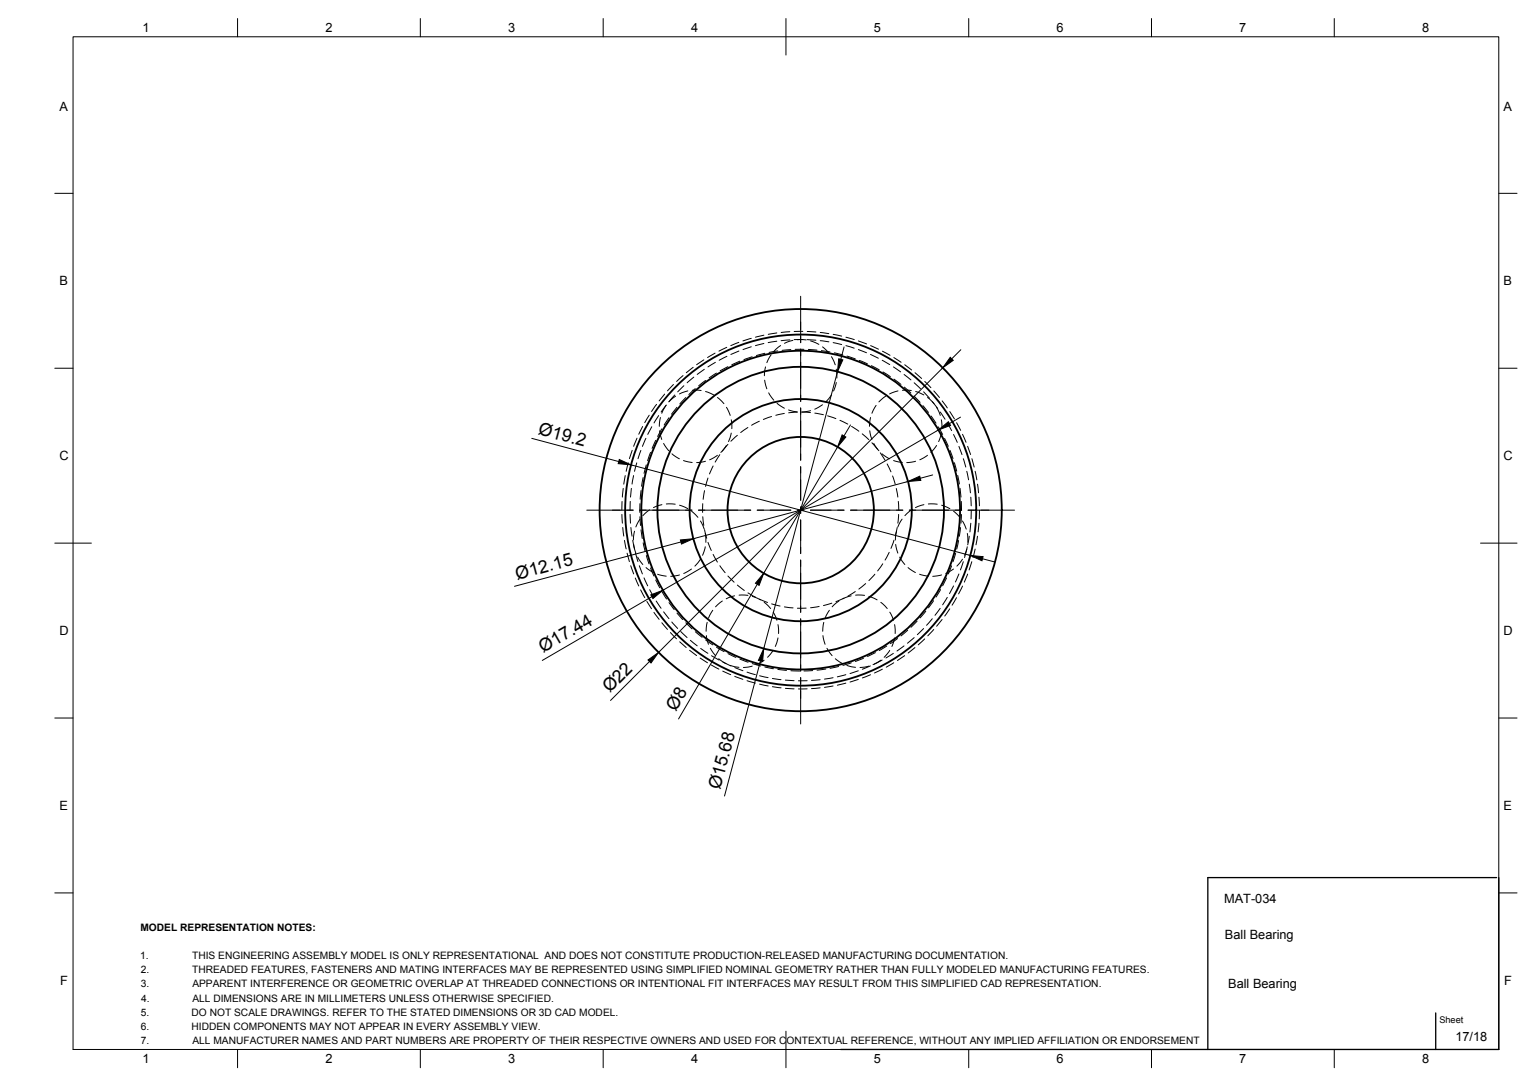
ISO-10303-21;
HEADER;
/* Generated by software containing ST-Developer
 * from STEP Tools, Inc. (www.steptools.com) 
 */

FILE_DESCRIPTION(
/* description */ ('STEP AP214'),
/* implementation_level */ '2;1');

FILE_NAME(
/* name */ 'Ball Bearing.step',
/* time_stamp */ '2026-11-14T09:24:36-08:00',
/* author */ (''),
/* organization */ (''),
/* preprocessor_version */ 'ST-DEVELOPER v20.2',
/* originating_system */ 'Autodesk Translation Framework v15.17.0.0',
/* authorisation */ '');

FILE_SCHEMA (('AUTOMOTIVE_DESIGN { 1 0 10303 214 3 1 1 }'));
ENDSEC;

DATA;
#10=MECHANICAL_DESIGN_GEOMETRIC_PRESENTATION_REPRESENTATION('',(#218,#219,#220,#221,#222,#223,#224,#225,#226),#18867);
#123=SPHERICAL_SURFACE('',#12164,1.9845);
#124=SPHERICAL_SURFACE('',#12166,1.9845);
#125=SPHERICAL_SURFACE('',#12168,1.9845);
#126=SPHERICAL_SURFACE('',#12170,1.9845);
#127=SPHERICAL_SURFACE('',#12172,1.9845);
#128=SPHERICAL_SURFACE('',#12174,1.9845);
#129=SPHERICAL_SURFACE('',#12176,1.9845);
#132=CONICAL_SURFACE('',#12193,8.8,1.39626340159546);
#133=CONICAL_SURFACE('',#12203,9.6,1.39626340159547);
#134=CONICAL_SURFACE('',#12217,9.6,1.46902152746005);
#135=CONICAL_SURFACE('',#12222,8.71875,1.51977681092793);
#136=CONICAL_SURFACE('',#12225,7.8375,1.51977681092793);
#137=CONICAL_SURFACE('',#12227,7.8375,1.51977681092793);
#138=CONICAL_SURFACE('',#12231,8.71875,1.46902152746005);
#139=CONICAL_SURFACE('',#12235,6.075,1.51977681092793);
#140=CONICAL_SURFACE('',#12238,8.71875,1.51977681092792);
#141=CONICAL_SURFACE('',#12242,9.6,1.51977681092792);
#157=TOROIDAL_SURFACE('',#12178,10.7,0.3);
#158=TOROIDAL_SURFACE('',#12184,10.7,0.3);
#159=TOROIDAL_SURFACE('',#12190,9.6,0.18);
#160=TOROIDAL_SURFACE('',#12197,7.35,1.9845);
#161=TOROIDAL_SURFACE('',#12206,9.6,0.18);
#162=TOROIDAL_SURFACE('',#12213,7.35,1.9845);
#163=TOROIDAL_SURFACE('',#12250,5.975,0.1);
#164=TOROIDAL_SURFACE('',#12253,4.3,0.3);
#165=TOROIDAL_SURFACE('',#12259,4.3,0.3);
#166=TOROIDAL_SURFACE('',#12262,5.975,0.1);
#186=SHAPE_REPRESENTATION_RELATIONSHIP('SRR','None',#18950,#202);
#202=ADVANCED_BREP_SHAPE_REPRESENTATION('',(#242,#243,#244,#245,#246,#247,
#248,#249,#250),#18866);
#218=STYLED_ITEM('',(#19027),#242);
#219=STYLED_ITEM('',(#19027),#243);
#220=STYLED_ITEM('',(#19027),#244);
#221=STYLED_ITEM('',(#19027),#245);
#222=STYLED_ITEM('',(#19027),#246);
#223=STYLED_ITEM('',(#19027),#247);
#224=STYLED_ITEM('',(#19027),#248);
#225=STYLED_ITEM('',(#19027),#249);
#226=STYLED_ITEM('',(#19027),#250);
#242=MANIFOLD_SOLID_BREP('Body1',#10973);
#243=MANIFOLD_SOLID_BREP('Body2',#10974);
#244=MANIFOLD_SOLID_BREP('Body3',#10975);
#245=MANIFOLD_SOLID_BREP('Body4',#10976);
#246=MANIFOLD_SOLID_BREP('Body5',#10977);
#247=MANIFOLD_SOLID_BREP('Body6',#10978);
#248=MANIFOLD_SOLID_BREP('Body7',#10979);
#249=MANIFOLD_SOLID_BREP('Body8',#10980);
#250=MANIFOLD_SOLID_BREP('Body9',#10981);
#373=FACE_BOUND('',#2012,.T.);
#374=FACE_BOUND('',#2014,.T.);
#375=FACE_BOUND('',#2036,.T.);
#376=FACE_BOUND('',#2038,.T.);
#377=FACE_BOUND('',#2040,.T.);
#378=FACE_BOUND('',#2042,.T.);
#379=FACE_BOUND('',#2044,.T.);
#380=FACE_BOUND('',#2046,.T.);
#717=PLANE('',#12211);
#718=PLANE('',#12212);
#719=PLANE('',#12269);
#720=PLANE('',#12270);
#721=PLANE('',#12271);
#722=PLANE('',#12272);
#723=PLANE('',#12273);
#724=PLANE('',#12274);
#1274=FACE_OUTER_BOUND('',#1992,.T.);
#1275=FACE_OUTER_BOUND('',#1993,.T.);
#1276=FACE_OUTER_BOUND('',#1994,.T.);
#1277=FACE_OUTER_BOUND('',#1995,.T.);
#1278=FACE_OUTER_BOUND('',#1996,.T.);
#1279=FACE_OUTER_BOUND('',#1997,.T.);
#1280=FACE_OUTER_BOUND('',#1998,.T.);
#1281=FACE_OUTER_BOUND('',#1999,.T.);
#1282=FACE_OUTER_BOUND('',#2000,.T.);
#1283=FACE_OUTER_BOUND('',#2001,.T.);
#1284=FACE_OUTER_BOUND('',#2002,.T.);
#1285=FACE_OUTER_BOUND('',#2003,.T.);
#1286=FACE_OUTER_BOUND('',#2004,.T.);
#1287=FACE_OUTER_BOUND('',#2005,.T.);
#1288=FACE_OUTER_BOUND('',#2006,.T.);
#1289=FACE_OUTER_BOUND('',#2007,.T.);
#1290=FACE_OUTER_BOUND('',#2008,.T.);
#1291=FACE_OUTER_BOUND('',#2009,.T.);
#1292=FACE_OUTER_BOUND('',#2010,.T.);
#1293=FACE_OUTER_BOUND('',#2011,.T.);
#1294=FACE_OUTER_BOUND('',#2013,.T.);
#1295=FACE_OUTER_BOUND('',#2015,.T.);
#1296=FACE_OUTER_BOUND('',#2016,.T.);
#1297=FACE_OUTER_BOUND('',#2017,.T.);
#1298=FACE_OUTER_BOUND('',#2018,.T.);
#1299=FACE_OUTER_BOUND('',#2019,.T.);
#1300=FACE_OUTER_BOUND('',#2020,.T.);
#1301=FACE_OUTER_BOUND('',#2021,.T.);
#1302=FACE_OUTER_BOUND('',#2022,.T.);
#1303=FACE_OUTER_BOUND('',#2023,.T.);
#1304=FACE_OUTER_BOUND('',#2024,.T.);
#1305=FACE_OUTER_BOUND('',#2025,.T.);
#1306=FACE_OUTER_BOUND('',#2026,.T.);
#1307=FACE_OUTER_BOUND('',#2027,.T.);
#1308=FACE_OUTER_BOUND('',#2028,.T.);
#1309=FACE_OUTER_BOUND('',#2029,.T.);
#1310=FACE_OUTER_BOUND('',#2030,.T.);
#1311=FACE_OUTER_BOUND('',#2031,.T.);
#1312=FACE_OUTER_BOUND('',#2032,.T.);
#1313=FACE_OUTER_BOUND('',#2033,.T.);
#1314=FACE_OUTER_BOUND('',#2034,.T.);
#1315=FACE_OUTER_BOUND('',#2035,.T.);
#1316=FACE_OUTER_BOUND('',#2037,.T.);
#1317=FACE_OUTER_BOUND('',#2039,.T.);
#1318=FACE_OUTER_BOUND('',#2041,.T.);
#1319=FACE_OUTER_BOUND('',#2043,.T.);
#1320=FACE_OUTER_BOUND('',#2045,.T.);
#1992=EDGE_LOOP('',(#9978,#9979));
#1993=EDGE_LOOP('',(#9980,#9981));
#1994=EDGE_LOOP('',(#9982,#9983));
#1995=EDGE_LOOP('',(#9984,#9985));
#1996=EDGE_LOOP('',(#9986,#9987));
#1997=EDGE_LOOP('',(#9988,#9989));
#1998=EDGE_LOOP('',(#9990,#9991));
#1999=EDGE_LOOP('',(#9992,#9993,#9994,#9995));
#2000=EDGE_LOOP('',(#9996,#9997,#9998,#9999));
#2001=EDGE_LOOP('',(#10000,#10001,#10002,#10003));
#2002=EDGE_LOOP('',(#10004,#10005,#10006,#10007));
#2003=EDGE_LOOP('',(#10008,#10009,#10010,#10011));
#2004=EDGE_LOOP('',(#10012,#10013,#10014,#10015));
#2005=EDGE_LOOP('',(#10016,#10017,#10018,#10019));
#2006=EDGE_LOOP('',(#10020,#10021,#10022,#10023));
#2007=EDGE_LOOP('',(#10024,#10025,#10026,#10027,#10028));
#2008=EDGE_LOOP('',(#10029,#10030,#10031,#10032,#10033,#10034));
#2009=EDGE_LOOP('',(#10035,#10036,#10037,#10038,#10039));
#2010=EDGE_LOOP('',(#10040,#10041,#10042,#10043));
#2011=EDGE_LOOP('',(#10044));
#2012=EDGE_LOOP('',(#10045));
#2013=EDGE_LOOP('',(#10046));
#2014=EDGE_LOOP('',(#10047));
#2015=EDGE_LOOP('',(#10048,#10049,#10050,#10051));
#2016=EDGE_LOOP('',(#10052,#10053,#10054,#10055));
#2017=EDGE_LOOP('',(#10056,#10057,#10058,#10059));
#2018=EDGE_LOOP('',(#10060,#10061,#10062,#10063,#10064));
#2019=EDGE_LOOP('',(#10065,#10066,#10067,#10068,#10069));
#2020=EDGE_LOOP('',(#10070,#10071,#10072,#10073,#10074));
#2021=EDGE_LOOP('',(#10075,#10076,#10077,#10078,#10079));
#2022=EDGE_LOOP('',(#10080,#10081,#10082,#10083));
#2023=EDGE_LOOP('',(#10084,#10085,#10086,#10087,#10088));
#2024=EDGE_LOOP('',(#10089,#10090,#10091,#10092,#10093,#10094));
#2025=EDGE_LOOP('',(#10095,#10096,#10097,#10098,#10099,#10100));
#2026=EDGE_LOOP('',(#10101,#10102,#10103,#10104));
#2027=EDGE_LOOP('',(#10105,#10106,#10107,#10108));
#2028=EDGE_LOOP('',(#10109,#10110,#10111,#10112));
#2029=EDGE_LOOP('',(#10113,#10114,#10115,#10116));
#2030=EDGE_LOOP('',(#10117,#10118,#10119,#10120));
#2031=EDGE_LOOP('',(#10121,#10122,#10123,#10124));
#2032=EDGE_LOOP('',(#10125,#10126,#10127,#10128));
#2033=EDGE_LOOP('',(#10129,#10130,#10131,#10132));
#2034=EDGE_LOOP('',(#10133,#10134,#10135,#10136,#10137));
#2035=EDGE_LOOP('',(#10138));
#2036=EDGE_LOOP('',(#10139));
#2037=EDGE_LOOP('',(#10140));
#2038=EDGE_LOOP('',(#10141));
#2039=EDGE_LOOP('',(#10142));
#2040=EDGE_LOOP('',(#10143));
#2041=EDGE_LOOP('',(#10144));
#2042=EDGE_LOOP('',(#10145));
#2043=EDGE_LOOP('',(#10146));
#2044=EDGE_LOOP('',(#10147));
#2045=EDGE_LOOP('',(#10148));
#2046=EDGE_LOOP('',(#10149));
#3039=LINE('',#18647,#4053);
#3040=LINE('',#18656,#4054);
#3041=LINE('',#18665,#4055);
#3042=LINE('',#18669,#4056);
#3043=LINE('',#18679,#4057);
#3044=LINE('',#18682,#4058);
#3045=LINE('',#18693,#4059);
#3046=LINE('',#18706,#4060);
#3047=LINE('',#18711,#4061);
#3048=LINE('',#18717,#4062);
#3049=LINE('',#18720,#4063);
#3050=LINE('',#18727,#4064);
#3051=LINE('',#18735,#4065);
#3052=LINE('',#18742,#4066);
#3053=LINE('',#18750,#4067);
#3054=LINE('',#18754,#4068);
#3055=LINE('',#18759,#4069);
#3056=LINE('',#18761,#4070);
#3057=LINE('',#18766,#4071);
#3058=LINE('',#18781,#4072);
#3059=LINE('',#18795,#4073);
#3060=LINE('',#18797,#4074);
#4053=VECTOR('',#15345,11.);
#4054=VECTOR('',#15356,9.6);
#4055=VECTOR('',#15369,8.8);
#4056=VECTOR('',#15374,8.8);
#4057=VECTOR('',#15387,8.8);
#4058=VECTOR('',#15390,9.6);
#4059=VECTOR('',#15405,9.6);
#4060=VECTOR('',#15422,9.6);
#4061=VECTOR('',#15429,9.6);
#4062=VECTOR('',#15436,8.71875);
#4063=VECTOR('',#15439,7.8375);
#4064=VECTOR('',#15446,7.8375);
#4065=VECTOR('',#15455,8.71875);
#4066=VECTOR('',#15464,6.075);
#4067=VECTOR('',#15473,8.71875);
#4068=VECTOR('',#15478,9.6);
#4069=VECTOR('',#15485,9.6);
#4070=VECTOR('',#15488,6.075);
#4071=VECTOR('',#15493,6.075);
#4072=VECTOR('',#15514,4.);
#4073=VECTOR('',#15533,6.075);
#4074=VECTOR('',#15536,6.075);
#4510=CIRCLE('',#12165,1.9845);
#4511=CIRCLE('',#12167,1.9845);
#4512=CIRCLE('',#12169,1.9845);
#4513=CIRCLE('',#12171,1.9845);
#4514=CIRCLE('',#12173,1.9845);
#4515=CIRCLE('',#12175,1.9845);
#4516=CIRCLE('',#12177,1.9845);
#4517=CIRCLE('',#12179,11.);
#4518=CIRCLE('',#12180,0.3);
#4519=CIRCLE('',#12181,10.7);
#4520=CIRCLE('',#12183,11.);
#4521=CIRCLE('',#12185,10.7);
#4522=CIRCLE('',#12186,0.3);
#4523=CIRCLE('',#12188,9.6);
#4524=CIRCLE('',#12189,9.6);
#4525=CIRCLE('',#12191,9.6);
#4526=CIRCLE('',#12192,0.18);
#4527=CIRCLE('',#12194,8.8);
#4528=CIRCLE('',#12196,8.8);
#4529=CIRCLE('',#12198,8.8);
#4530=CIRCLE('',#12199,1.9845);
#4531=CIRCLE('',#12201,8.8);
#4532=CIRCLE('',#12202,8.8);
#4533=CIRCLE('',#12204,9.6);
#4534=CIRCLE('',#12205,9.6);
#4535=CIRCLE('',#12207,9.6);
#4536=CIRCLE('',#12208,0.18);
#4537=CIRCLE('',#12210,9.6);
#4538=CIRCLE('',#12214,6.075);
#4539=CIRCLE('',#12215,1.9845);
#4540=CIRCLE('',#12216,6.075);
#4541=CIRCLE('',#12218,9.6);
#4542=CIRCLE('',#12219,8.71875);
#4543=CIRCLE('',#12221,9.6);
#4544=CIRCLE('',#12223,8.71875);
#4545=CIRCLE('',#12224,8.71875);
#4546=CIRCLE('',#12226,7.8375);
#4547=CIRCLE('',#12228,6.075);
#4548=CIRCLE('',#12229,7.8375);
#4549=CIRCLE('',#12230,6.075);
#4550=CIRCLE('',#12232,9.6);
#4551=CIRCLE('',#12233,8.71875);
#4552=CIRCLE('',#12234,9.6);
#4553=CIRCLE('',#12236,6.075);
#4554=CIRCLE('',#12237,7.8375);
#4555=CIRCLE('',#12239,8.71875);
#4556=CIRCLE('',#12240,8.71875);
#4557=CIRCLE('',#12241,7.8375);
#4558=CIRCLE('',#12243,9.6);
#4559=CIRCLE('',#12244,9.6);
#4560=CIRCLE('',#12248,6.075);
#4561=CIRCLE('',#12249,6.075);
#4562=CIRCLE('',#12251,5.975);
#4563=CIRCLE('',#12252,0.1);
#4564=CIRCLE('',#12254,4.);
#4565=CIRCLE('',#12255,0.3);
#4566=CIRCLE('',#12256,4.3);
#4567=CIRCLE('',#12258,4.);
#4568=CIRCLE('',#12260,4.3);
#4569=CIRCLE('',#12261,0.3);
#4570=CIRCLE('',#12263,6.075);
#4571=CIRCLE('',#12264,0.1);
#4572=CIRCLE('',#12265,5.975);
#4573=CIRCLE('',#12267,6.075);
#5526=VERTEX_POINT('',#18611);
#5527=VERTEX_POINT('',#18612);
#5528=VERTEX_POINT('',#18615);
#5529=VERTEX_POINT('',#18616);
#5530=VERTEX_POINT('',#18619);
#5531=VERTEX_POINT('',#18620);
#5532=VERTEX_POINT('',#18623);
#5533=VERTEX_POINT('',#18624);
#5534=VERTEX_POINT('',#18627);
#5535=VERTEX_POINT('',#18628);
#5536=VERTEX_POINT('',#18631);
#5537=VERTEX_POINT('',#18632);
#5538=VERTEX_POINT('',#18635);
#5539=VERTEX_POINT('',#18636);
#5540=VERTEX_POINT('',#18639);
#5541=VERTEX_POINT('',#18641);
#5542=VERTEX_POINT('',#18645);
#5543=VERTEX_POINT('',#18649);
#5544=VERTEX_POINT('',#18653);
#5545=VERTEX_POINT('',#18655);
#5546=VERTEX_POINT('',#18659);
#5547=VERTEX_POINT('',#18663);
#5548=VERTEX_POINT('',#18667);
#5549=VERTEX_POINT('',#18671);
#5550=VERTEX_POINT('',#18675);
#5551=VERTEX_POINT('',#18676);
#5552=VERTEX_POINT('',#18681);
#5553=VERTEX_POINT('',#18683);
#5554=VERTEX_POINT('',#18687);
#5555=VERTEX_POINT('',#18691);
#5556=VERTEX_POINT('',#18697);
#5557=VERTEX_POINT('',#18699);
#5558=VERTEX_POINT('',#18703);
#5559=VERTEX_POINT('',#18705);
#5560=VERTEX_POINT('',#18709);
#5561=VERTEX_POINT('',#18713);
#5562=VERTEX_POINT('',#18714);
#5563=VERTEX_POINT('',#18719);
#5564=VERTEX_POINT('',#18723);
#5565=VERTEX_POINT('',#18724);
#5566=VERTEX_POINT('',#18726);
#5567=VERTEX_POINT('',#18731);
#5568=VERTEX_POINT('',#18732);
#5569=VERTEX_POINT('',#18734);
#5570=VERTEX_POINT('',#18739);
#5571=VERTEX_POINT('',#18741);
#5572=VERTEX_POINT('',#18745);
#5573=VERTEX_POINT('',#18746);
#5574=VERTEX_POINT('',#18749);
#5575=VERTEX_POINT('',#18753);
#5576=VERTEX_POINT('',#18755);
#5577=VERTEX_POINT('',#18763);
#5578=VERTEX_POINT('',#18765);
#5579=VERTEX_POINT('',#18769);
#5580=VERTEX_POINT('',#18773);
#5581=VERTEX_POINT('',#18775);
#5582=VERTEX_POINT('',#18779);
#5583=VERTEX_POINT('',#18783);
#5584=VERTEX_POINT('',#18787);
#5585=VERTEX_POINT('',#18789);
#5586=VERTEX_POINT('',#18793);
#7022=EDGE_CURVE('',#5526,#5527,#4510,.T.);
#7023=EDGE_CURVE('',#5528,#5529,#4511,.T.);
#7024=EDGE_CURVE('',#5530,#5531,#4512,.T.);
#7025=EDGE_CURVE('',#5532,#5533,#4513,.T.);
#7026=EDGE_CURVE('',#5534,#5535,#4514,.T.);
#7027=EDGE_CURVE('',#5536,#5537,#4515,.T.);
#7028=EDGE_CURVE('',#5538,#5539,#4516,.T.);
#7029=EDGE_CURVE('',#5540,#5540,#4517,.T.);
#7030=EDGE_CURVE('',#5540,#5541,#4518,.T.);
#7031=EDGE_CURVE('',#5541,#5541,#4519,.T.);
#7032=EDGE_CURVE('',#5542,#5542,#4520,.T.);
#7033=EDGE_CURVE('',#5542,#5540,#3039,.T.);
#7034=EDGE_CURVE('',#5543,#5543,#4521,.T.);
#7035=EDGE_CURVE('',#5543,#5542,#4522,.T.);
#7036=EDGE_CURVE('',#5544,#5544,#4523,.T.);
#7037=EDGE_CURVE('',#5544,#5545,#3040,.T.);
#7038=EDGE_CURVE('',#5545,#5545,#4524,.T.);
#7039=EDGE_CURVE('',#5546,#5546,#4525,.T.);
#7040=EDGE_CURVE('',#5546,#5544,#4526,.T.);
#7041=EDGE_CURVE('',#5547,#5547,#4527,.T.);
#7042=EDGE_CURVE('',#5547,#5546,#3041,.T.);
#7043=EDGE_CURVE('',#5548,#5548,#4528,.T.);
#7044=EDGE_CURVE('',#5548,#5547,#3042,.T.);
#7045=EDGE_CURVE('',#5549,#5549,#4529,.T.);
#7046=EDGE_CURVE('',#5549,#5548,#4530,.T.);
#7047=EDGE_CURVE('',#5550,#5551,#4531,.T.);
#7048=EDGE_CURVE('',#5551,#5550,#4532,.T.);
#7049=EDGE_CURVE('',#5551,#5549,#3043,.T.);
#7050=EDGE_CURVE('',#5550,#5552,#3044,.T.);
#7051=EDGE_CURVE('',#5553,#5552,#4533,.T.);
#7052=EDGE_CURVE('',#5552,#5553,#4534,.T.);
#7053=EDGE_CURVE('',#5554,#5554,#4535,.T.);
#7054=EDGE_CURVE('',#5554,#5553,#4536,.T.);
#7055=EDGE_CURVE('',#5555,#5555,#4537,.T.);
#7056=EDGE_CURVE('',#5555,#5554,#3045,.T.);
#7057=EDGE_CURVE('',#5556,#5556,#4538,.T.);
#7058=EDGE_CURVE('',#5556,#5557,#4539,.T.);
#7059=EDGE_CURVE('',#5557,#5557,#4540,.T.);
#7060=EDGE_CURVE('',#5558,#5558,#4541,.T.);
#7061=EDGE_CURVE('',#5558,#5559,#3046,.T.);
#7062=EDGE_CURVE('',#5559,#5559,#4542,.T.);
#7063=EDGE_CURVE('',#5560,#5560,#4543,.T.);
#7064=EDGE_CURVE('',#5560,#5558,#3047,.T.);
#7065=EDGE_CURVE('',#5561,#5562,#4544,.T.);
#7066=EDGE_CURVE('',#5562,#5561,#4545,.T.);
#7067=EDGE_CURVE('',#5562,#5560,#3048,.T.);
#7068=EDGE_CURVE('',#5561,#5563,#3049,.T.);
#7069=EDGE_CURVE('',#5563,#5563,#4546,.T.);
#7070=EDGE_CURVE('',#5564,#5565,#4547,.T.);
#7071=EDGE_CURVE('',#5565,#5566,#3050,.T.);
#7072=EDGE_CURVE('',#5566,#5566,#4548,.T.);
#7073=EDGE_CURVE('',#5565,#5564,#4549,.T.);
#7074=EDGE_CURVE('',#5567,#5568,#4550,.T.);
#7075=EDGE_CURVE('',#5568,#5569,#3051,.T.);
#7076=EDGE_CURVE('',#5569,#5569,#4551,.T.);
#7077=EDGE_CURVE('',#5568,#5567,#4552,.T.);
#7078=EDGE_CURVE('',#5570,#5570,#4553,.T.);
#7079=EDGE_CURVE('',#5570,#5571,#3052,.T.);
#7080=EDGE_CURVE('',#5571,#5571,#4554,.T.);
#7081=EDGE_CURVE('',#5572,#5573,#4555,.T.);
#7082=EDGE_CURVE('',#5573,#5572,#4556,.T.);
#7083=EDGE_CURVE('',#5573,#5574,#3053,.T.);
#7084=EDGE_CURVE('',#5574,#5574,#4557,.T.);
#7085=EDGE_CURVE('',#5572,#5575,#3054,.T.);
#7086=EDGE_CURVE('',#5576,#5575,#4558,.T.);
#7087=EDGE_CURVE('',#5575,#5576,#4559,.T.);
#7088=EDGE_CURVE('',#5567,#5576,#3055,.T.);
#7089=EDGE_CURVE('',#5557,#5570,#3056,.T.);
#7090=EDGE_CURVE('',#5577,#5577,#4560,.T.);
#7091=EDGE_CURVE('',#5577,#5578,#3057,.T.);
#7092=EDGE_CURVE('',#5578,#5578,#4561,.T.);
#7093=EDGE_CURVE('',#5579,#5579,#4562,.T.);
#7094=EDGE_CURVE('',#5579,#5577,#4563,.T.);
#7095=EDGE_CURVE('',#5580,#5580,#4564,.T.);
#7096=EDGE_CURVE('',#5580,#5581,#4565,.T.);
#7097=EDGE_CURVE('',#5581,#5581,#4566,.T.);
#7098=EDGE_CURVE('',#5582,#5582,#4567,.T.);
#7099=EDGE_CURVE('',#5582,#5580,#3058,.T.);
#7100=EDGE_CURVE('',#5583,#5583,#4568,.T.);
#7101=EDGE_CURVE('',#5583,#5582,#4569,.T.);
#7102=EDGE_CURVE('',#5584,#5584,#4570,.T.);
#7103=EDGE_CURVE('',#5584,#5585,#4571,.T.);
#7104=EDGE_CURVE('',#5585,#5585,#4572,.T.);
#7105=EDGE_CURVE('',#5586,#5586,#4573,.T.);
#7106=EDGE_CURVE('',#5586,#5584,#3059,.T.);
#7107=EDGE_CURVE('',#5564,#5556,#3060,.T.);
#9978=ORIENTED_EDGE('',*,*,#7022,.T.);
#9979=ORIENTED_EDGE('',*,*,#7022,.F.);
#9980=ORIENTED_EDGE('',*,*,#7023,.T.);
#9981=ORIENTED_EDGE('',*,*,#7023,.F.);
#9982=ORIENTED_EDGE('',*,*,#7024,.T.);
#9983=ORIENTED_EDGE('',*,*,#7024,.F.);
#9984=ORIENTED_EDGE('',*,*,#7025,.T.);
#9985=ORIENTED_EDGE('',*,*,#7025,.F.);
#9986=ORIENTED_EDGE('',*,*,#7026,.T.);
#9987=ORIENTED_EDGE('',*,*,#7026,.F.);
#9988=ORIENTED_EDGE('',*,*,#7027,.T.);
#9989=ORIENTED_EDGE('',*,*,#7027,.F.);
#9990=ORIENTED_EDGE('',*,*,#7028,.T.);
#9991=ORIENTED_EDGE('',*,*,#7028,.F.);
#9992=ORIENTED_EDGE('',*,*,#7029,.F.);
#9993=ORIENTED_EDGE('',*,*,#7030,.T.);
#9994=ORIENTED_EDGE('',*,*,#7031,.T.);
#9995=ORIENTED_EDGE('',*,*,#7030,.F.);
#9996=ORIENTED_EDGE('',*,*,#7032,.F.);
#9997=ORIENTED_EDGE('',*,*,#7033,.T.);
#9998=ORIENTED_EDGE('',*,*,#7029,.T.);
#9999=ORIENTED_EDGE('',*,*,#7033,.F.);
#10000=ORIENTED_EDGE('',*,*,#7034,.F.);
#10001=ORIENTED_EDGE('',*,*,#7035,.T.);
#10002=ORIENTED_EDGE('',*,*,#7032,.T.);
#10003=ORIENTED_EDGE('',*,*,#7035,.F.);
#10004=ORIENTED_EDGE('',*,*,#7036,.F.);
#10005=ORIENTED_EDGE('',*,*,#7037,.T.);
#10006=ORIENTED_EDGE('',*,*,#7038,.T.);
#10007=ORIENTED_EDGE('',*,*,#7037,.F.);
#10008=ORIENTED_EDGE('',*,*,#7039,.F.);
#10009=ORIENTED_EDGE('',*,*,#7040,.T.);
#10010=ORIENTED_EDGE('',*,*,#7036,.T.);
#10011=ORIENTED_EDGE('',*,*,#7040,.F.);
#10012=ORIENTED_EDGE('',*,*,#7041,.F.);
#10013=ORIENTED_EDGE('',*,*,#7042,.T.);
#10014=ORIENTED_EDGE('',*,*,#7039,.T.);
#10015=ORIENTED_EDGE('',*,*,#7042,.F.);
#10016=ORIENTED_EDGE('',*,*,#7043,.F.);
#10017=ORIENTED_EDGE('',*,*,#7044,.T.);
#10018=ORIENTED_EDGE('',*,*,#7041,.T.);
#10019=ORIENTED_EDGE('',*,*,#7044,.F.);
#10020=ORIENTED_EDGE('',*,*,#7045,.F.);
#10021=ORIENTED_EDGE('',*,*,#7046,.T.);
#10022=ORIENTED_EDGE('',*,*,#7043,.T.);
#10023=ORIENTED_EDGE('',*,*,#7046,.F.);
#10024=ORIENTED_EDGE('',*,*,#7047,.F.);
#10025=ORIENTED_EDGE('',*,*,#7048,.F.);
#10026=ORIENTED_EDGE('',*,*,#7049,.T.);
#10027=ORIENTED_EDGE('',*,*,#7045,.T.);
#10028=ORIENTED_EDGE('',*,*,#7049,.F.);
#10029=ORIENTED_EDGE('',*,*,#7047,.T.);
#10030=ORIENTED_EDGE('',*,*,#7048,.T.);
#10031=ORIENTED_EDGE('',*,*,#7050,.T.);
#10032=ORIENTED_EDGE('',*,*,#7051,.F.);
#10033=ORIENTED_EDGE('',*,*,#7052,.F.);
#10034=ORIENTED_EDGE('',*,*,#7050,.F.);
#10035=ORIENTED_EDGE('',*,*,#7053,.F.);
#10036=ORIENTED_EDGE('',*,*,#7054,.T.);
#10037=ORIENTED_EDGE('',*,*,#7051,.T.);
#10038=ORIENTED_EDGE('',*,*,#7052,.T.);
#10039=ORIENTED_EDGE('',*,*,#7054,.F.);
#10040=ORIENTED_EDGE('',*,*,#7055,.F.);
#10041=ORIENTED_EDGE('',*,*,#7056,.T.);
#10042=ORIENTED_EDGE('',*,*,#7053,.T.);
#10043=ORIENTED_EDGE('',*,*,#7056,.F.);
#10044=ORIENTED_EDGE('',*,*,#7031,.F.);
#10045=ORIENTED_EDGE('',*,*,#7055,.T.);
#10046=ORIENTED_EDGE('',*,*,#7034,.T.);
#10047=ORIENTED_EDGE('',*,*,#7038,.F.);
#10048=ORIENTED_EDGE('',*,*,#7057,.F.);
#10049=ORIENTED_EDGE('',*,*,#7058,.T.);
#10050=ORIENTED_EDGE('',*,*,#7059,.T.);
#10051=ORIENTED_EDGE('',*,*,#7058,.F.);
#10052=ORIENTED_EDGE('',*,*,#7060,.F.);
#10053=ORIENTED_EDGE('',*,*,#7061,.T.);
#10054=ORIENTED_EDGE('',*,*,#7062,.T.);
#10055=ORIENTED_EDGE('',*,*,#7061,.F.);
#10056=ORIENTED_EDGE('',*,*,#7063,.F.);
#10057=ORIENTED_EDGE('',*,*,#7064,.T.);
#10058=ORIENTED_EDGE('',*,*,#7060,.T.);
#10059=ORIENTED_EDGE('',*,*,#7064,.F.);
#10060=ORIENTED_EDGE('',*,*,#7065,.F.);
#10061=ORIENTED_EDGE('',*,*,#7066,.F.);
#10062=ORIENTED_EDGE('',*,*,#7067,.T.);
#10063=ORIENTED_EDGE('',*,*,#7063,.T.);
#10064=ORIENTED_EDGE('',*,*,#7067,.F.);
#10065=ORIENTED_EDGE('',*,*,#7065,.T.);
#10066=ORIENTED_EDGE('',*,*,#7066,.T.);
#10067=ORIENTED_EDGE('',*,*,#7068,.T.);
#10068=ORIENTED_EDGE('',*,*,#7069,.F.);
#10069=ORIENTED_EDGE('',*,*,#7068,.F.);
#10070=ORIENTED_EDGE('',*,*,#7070,.T.);
#10071=ORIENTED_EDGE('',*,*,#7071,.T.);
#10072=ORIENTED_EDGE('',*,*,#7072,.F.);
#10073=ORIENTED_EDGE('',*,*,#7071,.F.);
#10074=ORIENTED_EDGE('',*,*,#7073,.T.);
#10075=ORIENTED_EDGE('',*,*,#7074,.T.);
#10076=ORIENTED_EDGE('',*,*,#7075,.T.);
#10077=ORIENTED_EDGE('',*,*,#7076,.F.);
#10078=ORIENTED_EDGE('',*,*,#7075,.F.);
#10079=ORIENTED_EDGE('',*,*,#7077,.T.);
#10080=ORIENTED_EDGE('',*,*,#7078,.F.);
#10081=ORIENTED_EDGE('',*,*,#7079,.T.);
#10082=ORIENTED_EDGE('',*,*,#7080,.T.);
#10083=ORIENTED_EDGE('',*,*,#7079,.F.);
#10084=ORIENTED_EDGE('',*,*,#7081,.F.);
#10085=ORIENTED_EDGE('',*,*,#7082,.F.);
#10086=ORIENTED_EDGE('',*,*,#7083,.T.);
#10087=ORIENTED_EDGE('',*,*,#7084,.T.);
#10088=ORIENTED_EDGE('',*,*,#7083,.F.);
#10089=ORIENTED_EDGE('',*,*,#7081,.T.);
#10090=ORIENTED_EDGE('',*,*,#7082,.T.);
#10091=ORIENTED_EDGE('',*,*,#7085,.T.);
#10092=ORIENTED_EDGE('',*,*,#7086,.F.);
#10093=ORIENTED_EDGE('',*,*,#7087,.F.);
#10094=ORIENTED_EDGE('',*,*,#7085,.F.);
#10095=ORIENTED_EDGE('',*,*,#7074,.F.);
#10096=ORIENTED_EDGE('',*,*,#7088,.T.);
#10097=ORIENTED_EDGE('',*,*,#7086,.T.);
#10098=ORIENTED_EDGE('',*,*,#7087,.T.);
#10099=ORIENTED_EDGE('',*,*,#7088,.F.);
#10100=ORIENTED_EDGE('',*,*,#7077,.F.);
#10101=ORIENTED_EDGE('',*,*,#7059,.F.);
#10102=ORIENTED_EDGE('',*,*,#7089,.T.);
#10103=ORIENTED_EDGE('',*,*,#7078,.T.);
#10104=ORIENTED_EDGE('',*,*,#7089,.F.);
#10105=ORIENTED_EDGE('',*,*,#7090,.F.);
#10106=ORIENTED_EDGE('',*,*,#7091,.T.);
#10107=ORIENTED_EDGE('',*,*,#7092,.T.);
#10108=ORIENTED_EDGE('',*,*,#7091,.F.);
#10109=ORIENTED_EDGE('',*,*,#7093,.F.);
#10110=ORIENTED_EDGE('',*,*,#7094,.T.);
#10111=ORIENTED_EDGE('',*,*,#7090,.T.);
#10112=ORIENTED_EDGE('',*,*,#7094,.F.);
#10113=ORIENTED_EDGE('',*,*,#7095,.F.);
#10114=ORIENTED_EDGE('',*,*,#7096,.T.);
#10115=ORIENTED_EDGE('',*,*,#7097,.T.);
#10116=ORIENTED_EDGE('',*,*,#7096,.F.);
#10117=ORIENTED_EDGE('',*,*,#7098,.F.);
#10118=ORIENTED_EDGE('',*,*,#7099,.T.);
#10119=ORIENTED_EDGE('',*,*,#7095,.T.);
#10120=ORIENTED_EDGE('',*,*,#7099,.F.);
#10121=ORIENTED_EDGE('',*,*,#7100,.F.);
#10122=ORIENTED_EDGE('',*,*,#7101,.T.);
#10123=ORIENTED_EDGE('',*,*,#7098,.T.);
#10124=ORIENTED_EDGE('',*,*,#7101,.F.);
#10125=ORIENTED_EDGE('',*,*,#7102,.F.);
#10126=ORIENTED_EDGE('',*,*,#7103,.T.);
#10127=ORIENTED_EDGE('',*,*,#7104,.T.);
#10128=ORIENTED_EDGE('',*,*,#7103,.F.);
#10129=ORIENTED_EDGE('',*,*,#7105,.F.);
#10130=ORIENTED_EDGE('',*,*,#7106,.T.);
#10131=ORIENTED_EDGE('',*,*,#7102,.T.);
#10132=ORIENTED_EDGE('',*,*,#7106,.F.);
#10133=ORIENTED_EDGE('',*,*,#7070,.F.);
#10134=ORIENTED_EDGE('',*,*,#7107,.T.);
#10135=ORIENTED_EDGE('',*,*,#7057,.T.);
#10136=ORIENTED_EDGE('',*,*,#7107,.F.);
#10137=ORIENTED_EDGE('',*,*,#7073,.F.);
#10138=ORIENTED_EDGE('',*,*,#7104,.F.);
#10139=ORIENTED_EDGE('',*,*,#7100,.T.);
#10140=ORIENTED_EDGE('',*,*,#7093,.T.);
#10141=ORIENTED_EDGE('',*,*,#7097,.F.);
#10142=ORIENTED_EDGE('',*,*,#7084,.F.);
#10143=ORIENTED_EDGE('',*,*,#7105,.T.);
#10144=ORIENTED_EDGE('',*,*,#7076,.T.);
#10145=ORIENTED_EDGE('',*,*,#7080,.F.);
#10146=ORIENTED_EDGE('',*,*,#7062,.F.);
#10147=ORIENTED_EDGE('',*,*,#7072,.T.);
#10148=ORIENTED_EDGE('',*,*,#7069,.T.);
#10149=ORIENTED_EDGE('',*,*,#7092,.F.);
#10350=CYLINDRICAL_SURFACE('',#12182,11.);
#10351=CYLINDRICAL_SURFACE('',#12187,9.6);
#10352=CYLINDRICAL_SURFACE('',#12195,8.8);
#10353=CYLINDRICAL_SURFACE('',#12200,8.8);
#10354=CYLINDRICAL_SURFACE('',#12209,9.6);
#10355=CYLINDRICAL_SURFACE('',#12220,9.6);
#10356=CYLINDRICAL_SURFACE('',#12245,9.6);
#10357=CYLINDRICAL_SURFACE('',#12246,6.075);
#10358=CYLINDRICAL_SURFACE('',#12247,6.075);
#10359=CYLINDRICAL_SURFACE('',#12257,4.);
#10360=CYLINDRICAL_SURFACE('',#12266,6.075);
#10361=CYLINDRICAL_SURFACE('',#12268,6.075);
#10911=ADVANCED_FACE('',(#1274),#123,.T.);
#10912=ADVANCED_FACE('',(#1275),#124,.T.);
#10913=ADVANCED_FACE('',(#1276),#125,.T.);
#10914=ADVANCED_FACE('',(#1277),#126,.T.);
#10915=ADVANCED_FACE('',(#1278),#127,.T.);
#10916=ADVANCED_FACE('',(#1279),#128,.T.);
#10917=ADVANCED_FACE('',(#1280),#129,.T.);
#10918=ADVANCED_FACE('',(#1281),#157,.T.);
#10919=ADVANCED_FACE('',(#1282),#10350,.T.);
#10920=ADVANCED_FACE('',(#1283),#158,.T.);
#10921=ADVANCED_FACE('',(#1284),#10351,.F.);
#10922=ADVANCED_FACE('',(#1285),#159,.F.);
#10923=ADVANCED_FACE('',(#1286),#132,.F.);
#10924=ADVANCED_FACE('',(#1287),#10352,.F.);
#10925=ADVANCED_FACE('',(#1288),#160,.F.);
#10926=ADVANCED_FACE('',(#1289),#10353,.F.);
#10927=ADVANCED_FACE('',(#1290),#133,.F.);
#10928=ADVANCED_FACE('',(#1291),#161,.F.);
#10929=ADVANCED_FACE('',(#1292),#10354,.F.);
#10930=ADVANCED_FACE('',(#1293,#373),#717,.T.);
#10931=ADVANCED_FACE('',(#1294,#374),#718,.T.);
#10932=ADVANCED_FACE('',(#1295),#162,.F.);
#10933=ADVANCED_FACE('',(#1296),#134,.T.);
#10934=ADVANCED_FACE('',(#1297),#10355,.T.);
#10935=ADVANCED_FACE('',(#1298),#135,.F.);
#10936=ADVANCED_FACE('',(#1299),#136,.T.);
#10937=ADVANCED_FACE('',(#1300),#137,.F.);
#10938=ADVANCED_FACE('',(#1301),#138,.T.);
#10939=ADVANCED_FACE('',(#1302),#139,.F.);
#10940=ADVANCED_FACE('',(#1303),#140,.T.);
#10941=ADVANCED_FACE('',(#1304),#141,.F.);
#10942=ADVANCED_FACE('',(#1305),#10356,.T.);
#10943=ADVANCED_FACE('',(#1306),#10357,.T.);
#10944=ADVANCED_FACE('',(#1307),#10358,.T.);
#10945=ADVANCED_FACE('',(#1308),#163,.T.);
#10946=ADVANCED_FACE('',(#1309),#164,.T.);
#10947=ADVANCED_FACE('',(#1310),#10359,.F.);
#10948=ADVANCED_FACE('',(#1311),#165,.T.);
#10949=ADVANCED_FACE('',(#1312),#166,.T.);
#10950=ADVANCED_FACE('',(#1313),#10360,.T.);
#10951=ADVANCED_FACE('',(#1314),#10361,.T.);
#10952=ADVANCED_FACE('',(#1315,#375),#719,.T.);
#10953=ADVANCED_FACE('',(#1316,#376),#720,.T.);
#10954=ADVANCED_FACE('',(#1317,#377),#721,.T.);
#10955=ADVANCED_FACE('',(#1318,#378),#722,.T.);
#10956=ADVANCED_FACE('',(#1319,#379),#723,.T.);
#10957=ADVANCED_FACE('',(#1320,#380),#724,.T.);
#10973=CLOSED_SHELL('',(#10911));
#10974=CLOSED_SHELL('',(#10912));
#10975=CLOSED_SHELL('',(#10913));
#10976=CLOSED_SHELL('',(#10914));
#10977=CLOSED_SHELL('',(#10915));
#10978=CLOSED_SHELL('',(#10916));
#10979=CLOSED_SHELL('',(#10917));
#10980=CLOSED_SHELL('',(#10918,#10919,#10920,#10921,#10922,#10923,#10924,
#10925,#10926,#10927,#10928,#10929,#10930,#10931));
#10981=CLOSED_SHELL('',(#10932,#10933,#10934,#10935,#10936,#10937,#10938,
#10939,#10940,#10941,#10942,#10943,#10944,#10945,#10946,#10947,#10948,#10949,
#10950,#10951,#10952,#10953,#10954,#10955,#10956,#10957));
#12163=AXIS2_PLACEMENT_3D('',#18609,#15303,#15304);
#12164=AXIS2_PLACEMENT_3D('',#18610,#15305,#15306);
#12165=AXIS2_PLACEMENT_3D('',#18613,#15307,#15308);
#12166=AXIS2_PLACEMENT_3D('',#18614,#15309,#15310);
#12167=AXIS2_PLACEMENT_3D('',#18617,#15311,#15312);
#12168=AXIS2_PLACEMENT_3D('',#18618,#15313,#15314);
#12169=AXIS2_PLACEMENT_3D('',#18621,#15315,#15316);
#12170=AXIS2_PLACEMENT_3D('',#18622,#15317,#15318);
#12171=AXIS2_PLACEMENT_3D('',#18625,#15319,#15320);
#12172=AXIS2_PLACEMENT_3D('',#18626,#15321,#15322);
#12173=AXIS2_PLACEMENT_3D('',#18629,#15323,#15324);
#12174=AXIS2_PLACEMENT_3D('',#18630,#15325,#15326);
#12175=AXIS2_PLACEMENT_3D('',#18633,#15327,#15328);
#12176=AXIS2_PLACEMENT_3D('',#18634,#15329,#15330);
#12177=AXIS2_PLACEMENT_3D('',#18637,#15331,#15332);
#12178=AXIS2_PLACEMENT_3D('',#18638,#15333,#15334);
#12179=AXIS2_PLACEMENT_3D('',#18640,#15335,#15336);
#12180=AXIS2_PLACEMENT_3D('',#18642,#15337,#15338);
#12181=AXIS2_PLACEMENT_3D('',#18643,#15339,#15340);
#12182=AXIS2_PLACEMENT_3D('',#18644,#15341,#15342);
#12183=AXIS2_PLACEMENT_3D('',#18646,#15343,#15344);
#12184=AXIS2_PLACEMENT_3D('',#18648,#15346,#15347);
#12185=AXIS2_PLACEMENT_3D('',#18650,#15348,#15349);
#12186=AXIS2_PLACEMENT_3D('',#18651,#15350,#15351);
#12187=AXIS2_PLACEMENT_3D('',#18652,#15352,#15353);
#12188=AXIS2_PLACEMENT_3D('',#18654,#15354,#15355);
#12189=AXIS2_PLACEMENT_3D('',#18657,#15357,#15358);
#12190=AXIS2_PLACEMENT_3D('',#18658,#15359,#15360);
#12191=AXIS2_PLACEMENT_3D('',#18660,#15361,#15362);
#12192=AXIS2_PLACEMENT_3D('',#18661,#15363,#15364);
#12193=AXIS2_PLACEMENT_3D('',#18662,#15365,#15366);
#12194=AXIS2_PLACEMENT_3D('',#18664,#15367,#15368);
#12195=AXIS2_PLACEMENT_3D('',#18666,#15370,#15371);
#12196=AXIS2_PLACEMENT_3D('',#18668,#15372,#15373);
#12197=AXIS2_PLACEMENT_3D('',#18670,#15375,#15376);
#12198=AXIS2_PLACEMENT_3D('',#18672,#15377,#15378);
#12199=AXIS2_PLACEMENT_3D('',#18673,#15379,#15380);
#12200=AXIS2_PLACEMENT_3D('',#18674,#15381,#15382);
#12201=AXIS2_PLACEMENT_3D('',#18677,#15383,#15384);
#12202=AXIS2_PLACEMENT_3D('',#18678,#15385,#15386);
#12203=AXIS2_PLACEMENT_3D('',#18680,#15388,#15389);
#12204=AXIS2_PLACEMENT_3D('',#18684,#15391,#15392);
#12205=AXIS2_PLACEMENT_3D('',#18685,#15393,#15394);
#12206=AXIS2_PLACEMENT_3D('',#18686,#15395,#15396);
#12207=AXIS2_PLACEMENT_3D('',#18688,#15397,#15398);
#12208=AXIS2_PLACEMENT_3D('',#18689,#15399,#15400);
#12209=AXIS2_PLACEMENT_3D('',#18690,#15401,#15402);
#12210=AXIS2_PLACEMENT_3D('',#18692,#15403,#15404);
#12211=AXIS2_PLACEMENT_3D('',#18694,#15406,#15407);
#12212=AXIS2_PLACEMENT_3D('',#18695,#15408,#15409);
#12213=AXIS2_PLACEMENT_3D('',#18696,#15410,#15411);
#12214=AXIS2_PLACEMENT_3D('',#18698,#15412,#15413);
#12215=AXIS2_PLACEMENT_3D('',#18700,#15414,#15415);
#12216=AXIS2_PLACEMENT_3D('',#18701,#15416,#15417);
#12217=AXIS2_PLACEMENT_3D('',#18702,#15418,#15419);
#12218=AXIS2_PLACEMENT_3D('',#18704,#15420,#15421);
#12219=AXIS2_PLACEMENT_3D('',#18707,#15423,#15424);
#12220=AXIS2_PLACEMENT_3D('',#18708,#15425,#15426);
#12221=AXIS2_PLACEMENT_3D('',#18710,#15427,#15428);
#12222=AXIS2_PLACEMENT_3D('',#18712,#15430,#15431);
#12223=AXIS2_PLACEMENT_3D('',#18715,#15432,#15433);
#12224=AXIS2_PLACEMENT_3D('',#18716,#15434,#15435);
#12225=AXIS2_PLACEMENT_3D('',#18718,#15437,#15438);
#12226=AXIS2_PLACEMENT_3D('',#18721,#15440,#15441);
#12227=AXIS2_PLACEMENT_3D('',#18722,#15442,#15443);
#12228=AXIS2_PLACEMENT_3D('',#18725,#15444,#15445);
#12229=AXIS2_PLACEMENT_3D('',#18728,#15447,#15448);
#12230=AXIS2_PLACEMENT_3D('',#18729,#15449,#15450);
#12231=AXIS2_PLACEMENT_3D('',#18730,#15451,#15452);
#12232=AXIS2_PLACEMENT_3D('',#18733,#15453,#15454);
#12233=AXIS2_PLACEMENT_3D('',#18736,#15456,#15457);
#12234=AXIS2_PLACEMENT_3D('',#18737,#15458,#15459);
#12235=AXIS2_PLACEMENT_3D('',#18738,#15460,#15461);
#12236=AXIS2_PLACEMENT_3D('',#18740,#15462,#15463);
#12237=AXIS2_PLACEMENT_3D('',#18743,#15465,#15466);
#12238=AXIS2_PLACEMENT_3D('',#18744,#15467,#15468);
#12239=AXIS2_PLACEMENT_3D('',#18747,#15469,#15470);
#12240=AXIS2_PLACEMENT_3D('',#18748,#15471,#15472);
#12241=AXIS2_PLACEMENT_3D('',#18751,#15474,#15475);
#12242=AXIS2_PLACEMENT_3D('',#18752,#15476,#15477);
#12243=AXIS2_PLACEMENT_3D('',#18756,#15479,#15480);
#12244=AXIS2_PLACEMENT_3D('',#18757,#15481,#15482);
#12245=AXIS2_PLACEMENT_3D('',#18758,#15483,#15484);
#12246=AXIS2_PLACEMENT_3D('',#18760,#15486,#15487);
#12247=AXIS2_PLACEMENT_3D('',#18762,#15489,#15490);
#12248=AXIS2_PLACEMENT_3D('',#18764,#15491,#15492);
#12249=AXIS2_PLACEMENT_3D('',#18767,#15494,#15495);
#12250=AXIS2_PLACEMENT_3D('',#18768,#15496,#15497);
#12251=AXIS2_PLACEMENT_3D('',#18770,#15498,#15499);
#12252=AXIS2_PLACEMENT_3D('',#18771,#15500,#15501);
#12253=AXIS2_PLACEMENT_3D('',#18772,#15502,#15503);
#12254=AXIS2_PLACEMENT_3D('',#18774,#15504,#15505);
#12255=AXIS2_PLACEMENT_3D('',#18776,#15506,#15507);
#12256=AXIS2_PLACEMENT_3D('',#18777,#15508,#15509);
#12257=AXIS2_PLACEMENT_3D('',#18778,#15510,#15511);
#12258=AXIS2_PLACEMENT_3D('',#18780,#15512,#15513);
#12259=AXIS2_PLACEMENT_3D('',#18782,#15515,#15516);
#12260=AXIS2_PLACEMENT_3D('',#18784,#15517,#15518);
#12261=AXIS2_PLACEMENT_3D('',#18785,#15519,#15520);
#12262=AXIS2_PLACEMENT_3D('',#18786,#15521,#15522);
#12263=AXIS2_PLACEMENT_3D('',#18788,#15523,#15524);
#12264=AXIS2_PLACEMENT_3D('',#18790,#15525,#15526);
#12265=AXIS2_PLACEMENT_3D('',#18791,#15527,#15528);
#12266=AXIS2_PLACEMENT_3D('',#18792,#15529,#15530);
#12267=AXIS2_PLACEMENT_3D('',#18794,#15531,#15532);
#12268=AXIS2_PLACEMENT_3D('',#18796,#15534,#15535);
#12269=AXIS2_PLACEMENT_3D('',#18798,#15537,#15538);
#12270=AXIS2_PLACEMENT_3D('',#18799,#15539,#15540);
#12271=AXIS2_PLACEMENT_3D('',#18800,#15541,#15542);
#12272=AXIS2_PLACEMENT_3D('',#18801,#15543,#15544);
#12273=AXIS2_PLACEMENT_3D('',#18802,#15545,#15546);
#12274=AXIS2_PLACEMENT_3D('',#18803,#15547,#15548);
#15303=DIRECTION('axis',(0.,0.,1.));
#15304=DIRECTION('refdir',(1.,0.,0.));
#15305=DIRECTION('center_axis',(0.,0.,-1.));
#15306=DIRECTION('ref_axis',(0.,1.,0.));
#15307=DIRECTION('center_axis',(-1.,0.,0.));
#15308=DIRECTION('ref_axis',(0.,-1.,0.));
#15309=DIRECTION('center_axis',(0.,1.1188944566643E-16,-1.));
#15310=DIRECTION('ref_axis',(0.,1.,0.));
#15311=DIRECTION('center_axis',(-1.,0.,0.));
#15312=DIRECTION('ref_axis',(0.,-1.,0.));
#15313=DIRECTION('center_axis',(0.,0.,-1.));
#15314=DIRECTION('ref_axis',(0.,1.,0.));
#15315=DIRECTION('center_axis',(-1.,0.,0.));
#15316=DIRECTION('ref_axis',(0.,-1.,0.));
#15317=DIRECTION('center_axis',(0.,0.,-1.));
#15318=DIRECTION('ref_axis',(0.,1.,0.));
#15319=DIRECTION('center_axis',(-1.,0.,0.));
#15320=DIRECTION('ref_axis',(0.,-1.,0.));
#15321=DIRECTION('center_axis',(0.,1.1188944566643E-16,-1.));
#15322=DIRECTION('ref_axis',(0.,1.,0.));
#15323=DIRECTION('center_axis',(-1.,0.,0.));
#15324=DIRECTION('ref_axis',(0.,-1.,0.));
#15325=DIRECTION('center_axis',(0.,0.,-1.));
#15326=DIRECTION('ref_axis',(0.,1.,0.));
#15327=DIRECTION('center_axis',(-1.,0.,0.));
#15328=DIRECTION('ref_axis',(0.,-1.,0.));
#15329=DIRECTION('center_axis',(0.,0.,-1.));
#15330=DIRECTION('ref_axis',(0.,1.,0.));
#15331=DIRECTION('center_axis',(-1.,0.,0.));
#15332=DIRECTION('ref_axis',(0.,-1.,0.));
#15333=DIRECTION('center_axis',(1.,0.,0.));
#15334=DIRECTION('ref_axis',(0.,0.,1.));
#15335=DIRECTION('center_axis',(1.,0.,0.));
#15336=DIRECTION('ref_axis',(0.,0.,1.));
#15337=DIRECTION('center_axis',(0.,1.,1.22464679914735E-16));
#15338=DIRECTION('ref_axis',(0.,1.22464679914735E-16,-1.));
#15339=DIRECTION('center_axis',(1.,0.,0.));
#15340=DIRECTION('ref_axis',(0.,0.,1.));
#15341=DIRECTION('center_axis',(1.,0.,0.));
#15342=DIRECTION('ref_axis',(0.,0.,1.));
#15343=DIRECTION('center_axis',(1.,0.,0.));
#15344=DIRECTION('ref_axis',(0.,0.,1.));
#15345=DIRECTION('',(-1.,0.,0.));
#15346=DIRECTION('center_axis',(1.,0.,0.));
#15347=DIRECTION('ref_axis',(0.,0.,1.));
#15348=DIRECTION('center_axis',(1.,0.,0.));
#15349=DIRECTION('ref_axis',(0.,0.,1.));
#15350=DIRECTION('center_axis',(0.,1.,1.22464679914735E-16));
#15351=DIRECTION('ref_axis',(0.,1.22464679914735E-16,-1.));
#15352=DIRECTION('center_axis',(1.,0.,0.));
#15353=DIRECTION('ref_axis',(0.,0.,1.));
#15354=DIRECTION('center_axis',(1.,0.,0.));
#15355=DIRECTION('ref_axis',(0.,0.,1.));
#15356=DIRECTION('',(1.,0.,0.));
#15357=DIRECTION('center_axis',(1.,0.,0.));
#15358=DIRECTION('ref_axis',(0.,0.,1.));
#15359=DIRECTION('center_axis',(1.,0.,0.));
#15360=DIRECTION('ref_axis',(0.,0.,1.));
#15361=DIRECTION('center_axis',(1.,0.,0.));
#15362=DIRECTION('ref_axis',(0.,0.,1.));
#15363=DIRECTION('center_axis',(0.,-1.,-1.22464679914735E-16));
#15364=DIRECTION('ref_axis',(0.,1.22464679914735E-16,-1.));
#15365=DIRECTION('center_axis',(1.,0.,0.));
#15366=DIRECTION('ref_axis',(0.,0.,1.));
#15367=DIRECTION('center_axis',(1.,0.,0.));
#15368=DIRECTION('ref_axis',(0.,0.,1.));
#15369=DIRECTION('',(0.173648177666934,1.2060416625019E-16,-0.984807753012207));
#15370=DIRECTION('center_axis',(1.,0.,0.));
#15371=DIRECTION('ref_axis',(0.,0.,1.));
#15372=DIRECTION('center_axis',(1.,0.,0.));
#15373=DIRECTION('ref_axis',(0.,0.,1.));
#15374=DIRECTION('',(1.,0.,0.));
#15375=DIRECTION('center_axis',(1.,0.,0.));
#15376=DIRECTION('ref_axis',(0.,0.,1.));
#15377=DIRECTION('center_axis',(1.,0.,0.));
#15378=DIRECTION('ref_axis',(0.,0.,1.));
#15379=DIRECTION('center_axis',(0.,-1.,-1.22464679914735E-16));
#15380=DIRECTION('ref_axis',(0.,1.22464679914735E-16,-1.));
#15381=DIRECTION('center_axis',(1.,0.,0.));
#15382=DIRECTION('ref_axis',(0.,0.,1.));
#15383=DIRECTION('center_axis',(1.,0.,0.));
#15384=DIRECTION('ref_axis',(0.,0.,1.));
#15385=DIRECTION('center_axis',(1.,0.,0.));
#15386=DIRECTION('ref_axis',(0.,0.,1.));
#15387=DIRECTION('',(1.,0.,0.));
#15388=DIRECTION('center_axis',(-1.,0.,0.));
#15389=DIRECTION('ref_axis',(0.,0.,-1.));
#15390=DIRECTION('',(-0.173648177666924,1.2060416625019E-16,0.984807753012209));
#15391=DIRECTION('center_axis',(1.,0.,0.));
#15392=DIRECTION('ref_axis',(0.,0.,1.));
#15393=DIRECTION('center_axis',(1.,0.,0.));
#15394=DIRECTION('ref_axis',(0.,0.,1.));
#15395=DIRECTION('center_axis',(1.,0.,0.));
#15396=DIRECTION('ref_axis',(0.,0.,1.));
#15397=DIRECTION('center_axis',(1.,0.,0.));
#15398=DIRECTION('ref_axis',(0.,0.,1.));
#15399=DIRECTION('center_axis',(0.,-1.,-1.22464679914735E-16));
#15400=DIRECTION('ref_axis',(0.,1.22464679914735E-16,-1.));
#15401=DIRECTION('center_axis',(1.,0.,0.));
#15402=DIRECTION('ref_axis',(0.,0.,1.));
#15403=DIRECTION('center_axis',(1.,0.,0.));
#15404=DIRECTION('ref_axis',(0.,0.,1.));
#15405=DIRECTION('',(1.,0.,0.));
#15406=DIRECTION('center_axis',(-1.,0.,0.));
#15407=DIRECTION('ref_axis',(0.,0.,-1.));
#15408=DIRECTION('center_axis',(1.,0.,0.));
#15409=DIRECTION('ref_axis',(0.,-1.,0.));
#15410=DIRECTION('center_axis',(1.,0.,0.));
#15411=DIRECTION('ref_axis',(0.,0.,1.));
#15412=DIRECTION('center_axis',(1.,0.,0.));
#15413=DIRECTION('ref_axis',(0.,0.,1.));
#15414=DIRECTION('center_axis',(0.,-1.,-1.22464679914735E-16));
#15415=DIRECTION('ref_axis',(0.,1.22464679914735E-16,-1.));
#15416=DIRECTION('center_axis',(1.,0.,0.));
#15417=DIRECTION('ref_axis',(0.,0.,1.));
#15418=DIRECTION('center_axis',(1.,0.,0.));
#15419=DIRECTION('ref_axis',(0.,0.,1.));
#15420=DIRECTION('center_axis',(1.,0.,0.));
#15421=DIRECTION('ref_axis',(0.,0.,1.));
#15422=DIRECTION('',(-0.101599191217213,-1.21830975896784E-16,0.994825414001878));
#15423=DIRECTION('center_axis',(1.,0.,0.));
#15424=DIRECTION('ref_axis',(0.,0.,1.));
#15425=DIRECTION('center_axis',(1.,0.,0.));
#15426=DIRECTION('ref_axis',(0.,0.,1.));
#15427=DIRECTION('center_axis',(1.,0.,0.));
#15428=DIRECTION('ref_axis',(0.,0.,1.));
#15429=DIRECTION('',(-1.,0.,0.));
#15430=DIRECTION('center_axis',(1.,0.,0.));
#15431=DIRECTION('ref_axis',(0.,0.,1.));
#15432=DIRECTION('center_axis',(1.,0.,0.));
#15433=DIRECTION('ref_axis',(0.,0.,1.));
#15434=DIRECTION('center_axis',(1.,0.,0.));
#15435=DIRECTION('ref_axis',(0.,0.,1.));
#15436=DIRECTION('',(0.0509973848574056,1.22305327255588E-16,-0.998698786790945));
#15437=DIRECTION('center_axis',(-1.,0.,0.));
#15438=DIRECTION('ref_axis',(0.,0.,-1.));
#15439=DIRECTION('',(0.0509973848574056,-1.22305327255588E-16,-0.998698786790945));
#15440=DIRECTION('center_axis',(1.,0.,0.));
#15441=DIRECTION('ref_axis',(0.,0.,1.));
#15442=DIRECTION('center_axis',(-1.,0.,0.));
#15443=DIRECTION('ref_axis',(0.,0.,-1.));
#15444=DIRECTION('center_axis',(1.,0.,0.));
#15445=DIRECTION('ref_axis',(0.,0.,1.));
#15446=DIRECTION('',(-0.0509973848574056,1.22305327255588E-16,0.998698786790945));
#15447=DIRECTION('center_axis',(1.,0.,0.));
#15448=DIRECTION('ref_axis',(0.,0.,1.));
#15449=DIRECTION('center_axis',(1.,0.,0.));
#15450=DIRECTION('ref_axis',(0.,0.,1.));
#15451=DIRECTION('center_axis',(-1.,0.,0.));
#15452=DIRECTION('ref_axis',(0.,0.,-1.));
#15453=DIRECTION('center_axis',(1.,0.,0.));
#15454=DIRECTION('ref_axis',(0.,0.,1.));
#15455=DIRECTION('',(0.101599191217213,-1.21830975896784E-16,-0.994825414001878));
#15456=DIRECTION('center_axis',(1.,0.,0.));
#15457=DIRECTION('ref_axis',(0.,0.,1.));
#15458=DIRECTION('center_axis',(1.,0.,0.));
#15459=DIRECTION('ref_axis',(0.,0.,1.));
#15460=DIRECTION('center_axis',(1.,0.,0.));
#15461=DIRECTION('ref_axis',(0.,0.,1.));
#15462=DIRECTION('center_axis',(1.,0.,0.));
#15463=DIRECTION('ref_axis',(0.,0.,1.));
#15464=DIRECTION('',(0.0509973848574056,1.22305327255588E-16,-0.998698786790945));
#15465=DIRECTION('center_axis',(1.,0.,0.));
#15466=DIRECTION('ref_axis',(0.,0.,1.));
#15467=DIRECTION('center_axis',(1.,0.,0.));
#15468=DIRECTION('ref_axis',(0.,0.,1.));
#15469=DIRECTION('center_axis',(1.,0.,0.));
#15470=DIRECTION('ref_axis',(0.,0.,1.));
#15471=DIRECTION('center_axis',(1.,0.,0.));
#15472=DIRECTION('ref_axis',(0.,0.,1.));
#15473=DIRECTION('',(-0.0509973848574156,-1.22305327255588E-16,0.998698786790945));
#15474=DIRECTION('center_axis',(1.,0.,0.));
#15475=DIRECTION('ref_axis',(0.,0.,1.));
#15476=DIRECTION('center_axis',(-1.,0.,0.));
#15477=DIRECTION('ref_axis',(0.,0.,-1.));
#15478=DIRECTION('',(-0.0509973848574156,1.22305327255587E-16,0.998698786790945));
#15479=DIRECTION('center_axis',(1.,0.,0.));
#15480=DIRECTION('ref_axis',(0.,0.,1.));
#15481=DIRECTION('center_axis',(1.,0.,0.));
#15482=DIRECTION('ref_axis',(0.,0.,1.));
#15483=DIRECTION('center_axis',(1.,0.,0.));
#15484=DIRECTION('ref_axis',(0.,0.,1.));
#15485=DIRECTION('',(-1.,0.,0.));
#15486=DIRECTION('center_axis',(1.,0.,0.));
#15487=DIRECTION('ref_axis',(0.,0.,1.));
#15488=DIRECTION('',(-1.,0.,0.));
#15489=DIRECTION('center_axis',(1.,0.,0.));
#15490=DIRECTION('ref_axis',(0.,0.,1.));
#15491=DIRECTION('center_axis',(1.,0.,0.));
#15492=DIRECTION('ref_axis',(0.,0.,1.));
#15493=DIRECTION('',(-1.,0.,0.));
#15494=DIRECTION('center_axis',(1.,0.,0.));
#15495=DIRECTION('ref_axis',(0.,0.,1.));
#15496=DIRECTION('center_axis',(1.,0.,0.));
#15497=DIRECTION('ref_axis',(0.,0.,1.));
#15498=DIRECTION('center_axis',(1.,0.,0.));
#15499=DIRECTION('ref_axis',(0.,0.,1.));
#15500=DIRECTION('center_axis',(0.,1.,1.22464679914735E-16));
#15501=DIRECTION('ref_axis',(0.,1.22464679914735E-16,-1.));
#15502=DIRECTION('center_axis',(1.,0.,0.));
#15503=DIRECTION('ref_axis',(0.,0.,1.));
#15504=DIRECTION('center_axis',(1.,0.,0.));
#15505=DIRECTION('ref_axis',(0.,0.,1.));
#15506=DIRECTION('center_axis',(0.,1.,1.22464679914735E-16));
#15507=DIRECTION('ref_axis',(0.,1.22464679914735E-16,-1.));
#15508=DIRECTION('center_axis',(1.,0.,0.));
#15509=DIRECTION('ref_axis',(0.,0.,1.));
#15510=DIRECTION('center_axis',(1.,0.,0.));
#15511=DIRECTION('ref_axis',(0.,0.,1.));
#15512=DIRECTION('center_axis',(1.,0.,0.));
#15513=DIRECTION('ref_axis',(0.,0.,1.));
#15514=DIRECTION('',(1.,0.,0.));
#15515=DIRECTION('center_axis',(1.,0.,0.));
#15516=DIRECTION('ref_axis',(0.,0.,1.));
#15517=DIRECTION('center_axis',(1.,0.,0.));
#15518=DIRECTION('ref_axis',(0.,0.,1.));
#15519=DIRECTION('center_axis',(0.,1.,1.22464679914735E-16));
#15520=DIRECTION('ref_axis',(0.,1.22464679914735E-16,-1.));
#15521=DIRECTION('center_axis',(1.,0.,0.));
#15522=DIRECTION('ref_axis',(0.,0.,1.));
#15523=DIRECTION('center_axis',(1.,0.,0.));
#15524=DIRECTION('ref_axis',(0.,0.,1.));
#15525=DIRECTION('center_axis',(0.,1.,1.22464679914735E-16));
#15526=DIRECTION('ref_axis',(0.,1.22464679914735E-16,-1.));
#15527=DIRECTION('center_axis',(1.,0.,0.));
#15528=DIRECTION('ref_axis',(0.,0.,1.));
#15529=DIRECTION('center_axis',(1.,0.,0.));
#15530=DIRECTION('ref_axis',(0.,0.,1.));
#15531=DIRECTION('center_axis',(1.,0.,0.));
#15532=DIRECTION('ref_axis',(0.,0.,1.));
#15533=DIRECTION('',(-1.,0.,0.));
#15534=DIRECTION('center_axis',(1.,0.,0.));
#15535=DIRECTION('ref_axis',(0.,0.,1.));
#15536=DIRECTION('',(-1.,0.,0.));
#15537=DIRECTION('center_axis',(-1.,0.,0.));
#15538=DIRECTION('ref_axis',(0.,0.,-1.));
#15539=DIRECTION('center_axis',(1.,0.,0.));
#15540=DIRECTION('ref_axis',(0.,-1.,0.));
#15541=DIRECTION('center_axis',(-1.,0.,0.));
#15542=DIRECTION('ref_axis',(0.,0.,-1.));
#15543=DIRECTION('center_axis',(1.,0.,0.));
#15544=DIRECTION('ref_axis',(0.,-1.,0.));
#15545=DIRECTION('center_axis',(-1.,0.,0.));
#15546=DIRECTION('ref_axis',(0.,0.,-1.));
#15547=DIRECTION('center_axis',(1.,0.,0.));
#15548=DIRECTION('ref_axis',(0.,-1.,0.));
#18609=CARTESIAN_POINT('',(0.,0.,0.));
#18610=CARTESIAN_POINT('Origin',(3.5,4.582650043662,-5.74646139614));
#18611=CARTESIAN_POINT('',(3.5,4.582650043662,-7.73096139614));
#18612=CARTESIAN_POINT('',(3.5,4.582650043662,-3.76196139614));
#18613=CARTESIAN_POINT('Origin',(3.5,4.582650043662,-5.74646139614));
#18614=CARTESIAN_POINT('Origin',(3.5,-1.635528864579,-7.165720154536));
#18615=CARTESIAN_POINT('',(3.5,-1.635528864579,-9.150220154536));
#18616=CARTESIAN_POINT('',(3.5,-1.635528864579,-5.181220154536));
#18617=CARTESIAN_POINT('Origin',(3.5,-1.635528864579,-7.165720154536));
#18618=CARTESIAN_POINT('Origin',(3.5,-6.622121179083,-3.189045482514));
#18619=CARTESIAN_POINT('',(3.5,-6.622121179083,-5.173545482514));
#18620=CARTESIAN_POINT('',(3.5,-6.622121179083,-1.204545482514));
#18621=CARTESIAN_POINT('Origin',(3.5,-6.622121179083,-3.189045482514));
#18622=CARTESIAN_POINT('Origin',(3.5,-6.622121179083,3.189045482514));
#18623=CARTESIAN_POINT('',(3.5,-6.622121179083,1.204545482514));
#18624=CARTESIAN_POINT('',(3.5,-6.622121179083,5.173545482514));
#18625=CARTESIAN_POINT('Origin',(3.5,-6.622121179083,3.189045482514));
#18626=CARTESIAN_POINT('Origin',(3.5,-1.635528864579,7.165720154536));
#18627=CARTESIAN_POINT('',(3.5,-1.635528864579,5.181220154536));
#18628=CARTESIAN_POINT('',(3.5,-1.635528864579,9.150220154536));
#18629=CARTESIAN_POINT('Origin',(3.5,-1.635528864579,7.165720154536));
#18630=CARTESIAN_POINT('Origin',(3.5,4.582650043662,5.74646139614));
#18631=CARTESIAN_POINT('',(3.5,4.582650043662,3.76196139614));
#18632=CARTESIAN_POINT('',(3.5,4.582650043662,7.73096139614));
#18633=CARTESIAN_POINT('Origin',(3.5,4.582650043662,5.74646139614));
#18634=CARTESIAN_POINT('Origin',(3.5,7.35,0.));
#18635=CARTESIAN_POINT('',(3.5,7.35,-1.9845));
#18636=CARTESIAN_POINT('',(3.5,7.35,1.9845));
#18637=CARTESIAN_POINT('Origin',(3.5,7.35,0.));
#18638=CARTESIAN_POINT('Origin',(0.3,0.,0.));
#18639=CARTESIAN_POINT('',(0.3,1.34711147906209E-15,-11.));
#18640=CARTESIAN_POINT('Origin',(0.3,0.,0.));
#18641=CARTESIAN_POINT('',(0.,1.31037207508767E-15,-10.7));
#18642=CARTESIAN_POINT('Origin',(0.3,1.31037207508767E-15,-10.7));
#18643=CARTESIAN_POINT('Origin',(0.,0.,0.));
#18644=CARTESIAN_POINT('Origin',(50.,0.,0.));
#18645=CARTESIAN_POINT('',(6.7,1.34711147906209E-15,-11.));
#18646=CARTESIAN_POINT('Origin',(6.7,0.,0.));
#18647=CARTESIAN_POINT('',(50.,1.34711147906209E-15,-11.));
#18648=CARTESIAN_POINT('Origin',(6.7,0.,0.));
#18649=CARTESIAN_POINT('',(7.,1.31037207508767E-15,-10.7));
#18650=CARTESIAN_POINT('Origin',(7.,0.,0.));
#18651=CARTESIAN_POINT('Origin',(6.7,1.31037207508767E-15,-10.7));
#18652=CARTESIAN_POINT('Origin',(50.,0.,0.));
#18653=CARTESIAN_POINT('',(6.91,1.17566092718146E-15,-9.6));
#18654=CARTESIAN_POINT('Origin',(6.91,0.,0.));
#18655=CARTESIAN_POINT('',(7.,1.17566092718146E-15,-9.6));
#18656=CARTESIAN_POINT('',(50.,1.17566092718146E-15,-9.6));
#18657=CARTESIAN_POINT('Origin',(7.,0.,0.));
#18658=CARTESIAN_POINT('Origin',(6.73,0.,0.));
#18659=CARTESIAN_POINT('',(6.55,1.17566092718146E-15,-9.6));
#18660=CARTESIAN_POINT('Origin',(6.55,0.,0.));
#18661=CARTESIAN_POINT('Origin',(6.73,1.17566092718146E-15,-9.6));
#18662=CARTESIAN_POINT('Origin',(6.40893841543323,0.,0.));
#18663=CARTESIAN_POINT('',(6.40893841543323,1.07768918324967E-15,-8.8));
#18664=CARTESIAN_POINT('Origin',(6.40893841543323,0.,0.));
#18665=CARTESIAN_POINT('',(6.40893841543323,1.07768918324967E-15,-8.8));
#18666=CARTESIAN_POINT('Origin',(50.,0.,0.));
#18667=CARTESIAN_POINT('',(4.85489492212496,1.07768918324967E-15,-8.8));
#18668=CARTESIAN_POINT('Origin',(4.85489492212496,0.,0.));
#18669=CARTESIAN_POINT('',(50.,1.07768918324967E-15,-8.8));
#18670=CARTESIAN_POINT('Origin',(3.5,0.,0.));
#18671=CARTESIAN_POINT('',(2.14510507787504,1.07768918324967E-15,-8.8));
#18672=CARTESIAN_POINT('Origin',(2.14510507787504,0.,0.));
#18673=CARTESIAN_POINT('Origin',(3.5,9.00115397373305E-16,-7.35));
#18674=CARTESIAN_POINT('Origin',(50.,0.,0.));
#18675=CARTESIAN_POINT('',(0.591061584566767,-1.12667505521557E-15,8.8));
#18676=CARTESIAN_POINT('',(0.59106158456677,1.07768918324967E-15,-8.8));
#18677=CARTESIAN_POINT('Origin',(0.591061584566767,0.,0.));
#18678=CARTESIAN_POINT('Origin',(0.591061584566767,0.,0.));
#18679=CARTESIAN_POINT('',(50.,1.07768918324967E-15,-8.8));
#18680=CARTESIAN_POINT('Origin',(0.45,0.,0.));
#18681=CARTESIAN_POINT('',(0.45,1.17566092718146E-15,9.6));
#18682=CARTESIAN_POINT('',(0.45,1.17566092718146E-15,9.6));
#18683=CARTESIAN_POINT('',(0.45,-1.17566092718146E-15,-9.6));
#18684=CARTESIAN_POINT('Origin',(0.45,0.,0.));
#18685=CARTESIAN_POINT('Origin',(0.45,0.,0.));
#18686=CARTESIAN_POINT('Origin',(0.27,0.,0.));
#18687=CARTESIAN_POINT('',(0.09,1.17566092718146E-15,-9.6));
#18688=CARTESIAN_POINT('Origin',(0.09,0.,0.));
#18689=CARTESIAN_POINT('Origin',(0.27,1.17566092718146E-15,-9.6));
#18690=CARTESIAN_POINT('Origin',(50.,0.,0.));
#18691=CARTESIAN_POINT('',(0.,1.17566092718146E-15,-9.6));
#18692=CARTESIAN_POINT('Origin',(0.,0.,0.));
#18693=CARTESIAN_POINT('',(50.,1.17566092718146E-15,-9.6));
#18694=CARTESIAN_POINT('Origin',(-3.25260651745651E-16,-10.7,0.));
#18695=CARTESIAN_POINT('Origin',(7.,-9.6,0.));
#18696=CARTESIAN_POINT('Origin',(3.5,0.,0.));
#18697=CARTESIAN_POINT('',(5.020728526069,-7.43972930482017E-16,-6.075));
#18698=CARTESIAN_POINT('Origin',(5.020728526069,0.,0.));
#18699=CARTESIAN_POINT('',(1.979271473931,7.43972930482017E-16,-6.075));
#18700=CARTESIAN_POINT('Origin',(3.5,9.00115397373305E-16,-7.35));
#18701=CARTESIAN_POINT('Origin',(1.979271473931,0.,0.));
#18702=CARTESIAN_POINT('Origin',(6.64,0.,0.));
#18703=CARTESIAN_POINT('',(6.64,1.17566092718146E-15,-9.6));
#18704=CARTESIAN_POINT('Origin',(6.64,0.,0.));
#18705=CARTESIAN_POINT('',(6.55,1.0677389280066E-15,-8.71875));
#18706=CARTESIAN_POINT('',(6.64,1.17566092718146E-15,-9.6));
#18707=CARTESIAN_POINT('Origin',(6.55,0.,0.));
#18708=CARTESIAN_POINT('Origin',(50.,0.,0.));
#18709=CARTESIAN_POINT('',(6.73,1.17566092718146E-15,-9.6));
#18710=CARTESIAN_POINT('Origin',(6.73,0.,0.));
#18711=CARTESIAN_POINT('',(50.,1.17566092718146E-15,-9.6));
#18712=CARTESIAN_POINT('Origin',(6.685,0.,0.));
#18713=CARTESIAN_POINT('',(6.685,-1.06773892800661E-15,8.71875000000007));
#18714=CARTESIAN_POINT('',(6.685,1.0677389280066E-15,-8.71875));
#18715=CARTESIAN_POINT('Origin',(6.685,0.,0.));
#18716=CARTESIAN_POINT('Origin',(6.685,0.,0.));
#18717=CARTESIAN_POINT('',(6.685,1.0677389280066E-15,-8.71875));
#18718=CARTESIAN_POINT('Origin',(6.73,0.,0.));
#18719=CARTESIAN_POINT('',(6.73,9.59816928831738E-16,7.8375));
#18720=CARTESIAN_POINT('',(6.73,9.59816928831738E-16,7.8375));
#18721=CARTESIAN_POINT('Origin',(6.73,0.,0.));
#18722=CARTESIAN_POINT('Origin',(6.55,0.,0.));
#18723=CARTESIAN_POINT('',(6.64,-7.43972930482017E-16,-6.075));
#18724=CARTESIAN_POINT('',(6.63999999999999,7.43972930482017E-16,6.075));
#18725=CARTESIAN_POINT('Origin',(6.64,0.,0.));
#18726=CARTESIAN_POINT('',(6.55,9.59816928831738E-16,7.8375));
#18727=CARTESIAN_POINT('',(6.55,9.59816928831738E-16,7.8375));
#18728=CARTESIAN_POINT('Origin',(6.55,0.,0.));
#18729=CARTESIAN_POINT('Origin',(6.64,0.,0.));
#18730=CARTESIAN_POINT('Origin',(0.45,0.,0.));
#18731=CARTESIAN_POINT('',(0.36,-1.17566092718146E-15,-9.6));
#18732=CARTESIAN_POINT('',(0.36,1.17566092718146E-15,9.6));
#18733=CARTESIAN_POINT('Origin',(0.36,0.,0.));
#18734=CARTESIAN_POINT('',(0.45,1.0677389280066E-15,8.71875));
#18735=CARTESIAN_POINT('',(0.45,1.0677389280066E-15,8.71875));
#18736=CARTESIAN_POINT('Origin',(0.45,0.,0.));
#18737=CARTESIAN_POINT('Origin',(0.36,0.,0.));
#18738=CARTESIAN_POINT('Origin',(0.36,0.,0.));
#18739=CARTESIAN_POINT('',(0.36,7.43972930482017E-16,-6.075));
#18740=CARTESIAN_POINT('Origin',(0.36,0.,0.));
#18741=CARTESIAN_POINT('',(0.449999999999993,9.59816928831738E-16,-7.8375));
#18742=CARTESIAN_POINT('',(0.36,7.43972930482017E-16,-6.075));
#18743=CARTESIAN_POINT('Origin',(0.45,0.,0.));
#18744=CARTESIAN_POINT('Origin',(0.315,0.,0.));
#18745=CARTESIAN_POINT('',(0.315,-1.12169992759403E-15,8.71875));
#18746=CARTESIAN_POINT('',(0.315,1.0677389280066E-15,-8.71875));
#18747=CARTESIAN_POINT('Origin',(0.315,0.,0.));
#18748=CARTESIAN_POINT('Origin',(0.315,0.,0.));
#18749=CARTESIAN_POINT('',(0.269999999999995,9.59816928831738E-16,-7.8375));
#18750=CARTESIAN_POINT('',(0.315,1.0677389280066E-15,-8.71875));
#18751=CARTESIAN_POINT('Origin',(0.27,0.,0.));
#18752=CARTESIAN_POINT('Origin',(0.27,0.,0.));
#18753=CARTESIAN_POINT('',(0.27,1.17566092718146E-15,9.6));
#18754=CARTESIAN_POINT('',(0.27,1.17566092718146E-15,9.6));
#18755=CARTESIAN_POINT('',(0.27,-1.17566092718146E-15,-9.6));
#18756=CARTESIAN_POINT('Origin',(0.27,0.,0.));
#18757=CARTESIAN_POINT('Origin',(0.27,0.,0.));
#18758=CARTESIAN_POINT('Origin',(50.,0.,0.));
#18759=CARTESIAN_POINT('',(50.,1.17566092718146E-15,-9.6));
#18760=CARTESIAN_POINT('Origin',(50.,0.,0.));
#18761=CARTESIAN_POINT('',(50.,7.43972930482017E-16,-6.075));
#18762=CARTESIAN_POINT('Origin',(50.,0.,0.));
#18763=CARTESIAN_POINT('',(6.9,7.43972930482017E-16,-6.075));
#18764=CARTESIAN_POINT('Origin',(6.9,0.,0.));
#18765=CARTESIAN_POINT('',(6.73,7.43972930482017E-16,-6.075));
#18766=CARTESIAN_POINT('',(50.,7.43972930482017E-16,-6.075));
#18767=CARTESIAN_POINT('Origin',(6.73,0.,0.));
#18768=CARTESIAN_POINT('Origin',(6.9,0.,0.));
#18769=CARTESIAN_POINT('',(7.,7.31726462490544E-16,-5.975));
#18770=CARTESIAN_POINT('Origin',(7.,0.,0.));
#18771=CARTESIAN_POINT('Origin',(6.9,7.31726462490544E-16,-5.975));
#18772=CARTESIAN_POINT('Origin',(6.7,0.,0.));
#18773=CARTESIAN_POINT('',(6.7,4.89858719658941E-16,-4.));
#18774=CARTESIAN_POINT('Origin',(6.7,0.,0.));
#18775=CARTESIAN_POINT('',(7.,5.26598123633362E-16,-4.3));
#18776=CARTESIAN_POINT('Origin',(6.7,5.26598123633362E-16,-4.3));
#18777=CARTESIAN_POINT('Origin',(7.,0.,0.));
#18778=CARTESIAN_POINT('Origin',(50.,0.,0.));
#18779=CARTESIAN_POINT('',(0.300000000000002,4.89858719658941E-16,-4.));
#18780=CARTESIAN_POINT('Origin',(0.3,0.,0.));
#18781=CARTESIAN_POINT('',(50.,4.89858719658941E-16,-4.));
#18782=CARTESIAN_POINT('Origin',(0.3,0.,0.));
#18783=CARTESIAN_POINT('',(0.,5.26598123633362E-16,-4.3));
#18784=CARTESIAN_POINT('Origin',(0.,0.,0.));
#18785=CARTESIAN_POINT('Origin',(0.3,5.26598123633362E-16,-4.3));
#18786=CARTESIAN_POINT('Origin',(0.1,0.,0.));
#18787=CARTESIAN_POINT('',(0.100000000000003,7.43972930482017E-16,-6.075));
#18788=CARTESIAN_POINT('Origin',(0.100000000000003,0.,0.));
#18789=CARTESIAN_POINT('',(0.,7.31726462490544E-16,-5.975));
#18790=CARTESIAN_POINT('Origin',(0.1,7.31726462490544E-16,-5.975));
#18791=CARTESIAN_POINT('Origin',(0.,0.,0.));
#18792=CARTESIAN_POINT('Origin',(50.,0.,0.));
#18793=CARTESIAN_POINT('',(0.27000000000001,7.43972930482017E-16,-6.075));
#18794=CARTESIAN_POINT('Origin',(0.27,0.,0.));
#18795=CARTESIAN_POINT('',(50.,7.43972930482017E-16,-6.075));
#18796=CARTESIAN_POINT('Origin',(50.,0.,0.));
#18797=CARTESIAN_POINT('',(50.,7.43972930482017E-16,-6.075));
#18798=CARTESIAN_POINT('Origin',(0.,-5.975,0.));
#18799=CARTESIAN_POINT('Origin',(7.,-4.3,0.));
#18800=CARTESIAN_POINT('Origin',(0.27,-7.8375,0.));
#18801=CARTESIAN_POINT('Origin',(0.45,-7.8375,0.));
#18802=CARTESIAN_POINT('Origin',(6.55,-8.71875,0.));
#18803=CARTESIAN_POINT('Origin',(6.73,-6.075,0.));
#18848=UNCERTAINTY_MEASURE_WITH_UNIT(LENGTH_MEASURE(0.01),#18868,
'DISTANCE_ACCURACY_VALUE',
'Maximum model space distance between geometric entities at asserted c
onnectivities');
#18849=UNCERTAINTY_MEASURE_WITH_UNIT(LENGTH_MEASURE(0.01),#18868,
'DISTANCE_ACCURACY_VALUE',
'Maximum model space distance between geometric entities at asserted c
onnectivities');
#18866=(
GEOMETRIC_REPRESENTATION_CONTEXT(3)
GLOBAL_UNCERTAINTY_ASSIGNED_CONTEXT((#18848))
GLOBAL_UNIT_ASSIGNED_CONTEXT((#18868,#18870,#18871))
REPRESENTATION_CONTEXT('','3D')
);
#18867=(
GEOMETRIC_REPRESENTATION_CONTEXT(3)
GLOBAL_UNCERTAINTY_ASSIGNED_CONTEXT((#18849))
GLOBAL_UNIT_ASSIGNED_CONTEXT((#18868,#18870,#18871))
REPRESENTATION_CONTEXT('','3D')
);
#18868=(
LENGTH_UNIT()
NAMED_UNIT(*)
SI_UNIT(.MILLI.,.METRE.)
);
#18870=(
NAMED_UNIT(*)
PLANE_ANGLE_UNIT()
SI_UNIT($,.RADIAN.)
);
#18871=(
NAMED_UNIT(*)
SI_UNIT($,.STERADIAN.)
SOLID_ANGLE_UNIT()
);
#18888=SHAPE_DEFINITION_REPRESENTATION(#18905,#18950);
#18905=PRODUCT_DEFINITION_SHAPE('',$,#18968);
#18950=SHAPE_REPRESENTATION('',(#12163),#18866);
#18951=PRODUCT_DEFINITION_CONTEXT('part definition',#19004,'design');
#18968=PRODUCT_DEFINITION('Ball Bearing','Ball Bearing',#18985,#18951);
#18985=PRODUCT_DEFINITION_FORMATION('',$,#19022);
#19004=APPLICATION_CONTEXT(
'Core Data for Automotive Mechanical Design Process');
#19005=PRODUCT_CONTEXT('part definition',#19004,'mechanical');
#19022=PRODUCT('Ball Bearing','Ball Bearing',$,(#19005));
#19027=PRESENTATION_STYLE_ASSIGNMENT((#19033));
#19033=SURFACE_STYLE_USAGE(.BOTH.,#19039);
#19039=SURFACE_SIDE_STYLE('',(#19045));
#19045=SURFACE_STYLE_FILL_AREA(#19051);
#19051=FILL_AREA_STYLE('Opaque(122,133,145)',(#19057));
#19057=FILL_AREA_STYLE_COLOUR('Opaque(122,133,145)',#19063);
#19063=COLOUR_RGB('Opaque(122,133,145)',0.47843137254902,0.52156862745098,
0.568627450980392);
ENDSEC;
END-ISO-10303-21;
